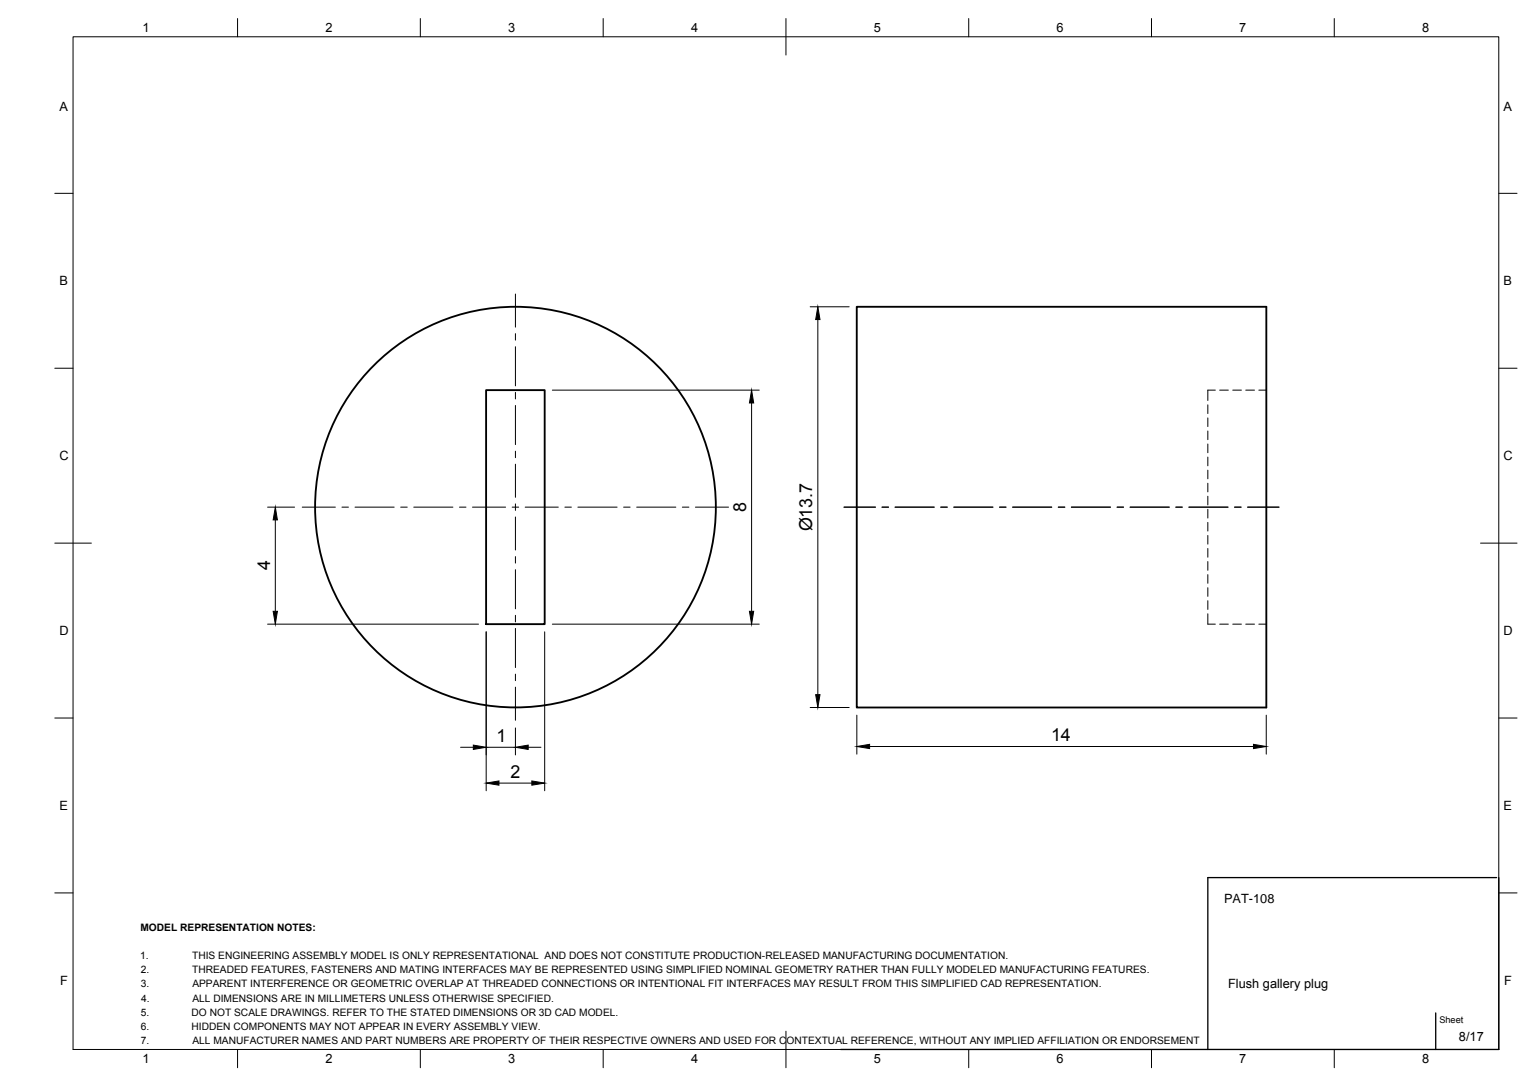
ISO-10303-21;
HEADER;
/* Generated by software containing ST-Developer
 * from STEP Tools, Inc. (www.steptools.com) 
 */

FILE_DESCRIPTION(
/* description */ ('Sub-base valve envelopes and connections'),
/* implementation_level */ '2;1');

FILE_NAME(
/* name */ 'Flush gallery plug.step',
/* time_stamp */ '2026-10-29T15:55:44-07:00',
/* author */ (''),
/* organization */ (''),
/* preprocessor_version */ 'ST-DEVELOPER v20.2',
/* originating_system */ 'Autodesk Translation Framework v15.17.0.0',
/* authorisation */ '');

FILE_SCHEMA (('AUTOMOTIVE_DESIGN { 1 0 10303 214 3 1 1 }'));
ENDSEC;

DATA;
#10=MECHANICAL_DESIGN_GEOMETRIC_PRESENTATION_REPRESENTATION('',(#124),#6113);
#100=SHAPE_REPRESENTATION_RELATIONSHIP('SRR','None',#6173,#112);
#112=ADVANCED_BREP_SHAPE_REPRESENTATION('',(#136),#6104);
#124=STYLED_ITEM('',(#6329),#136);
#136=MANIFOLD_SOLID_BREP('Body1',#3363);
#211=FACE_BOUND('',#762,.T.);
#326=PLANE('',#3711);
#327=PLANE('',#3712);
#328=PLANE('',#3713);
#329=PLANE('',#3714);
#330=PLANE('',#3715);
#331=PLANE('',#3716);
#332=PLANE('',#3720);
#488=FACE_OUTER_BOUND('',#756,.T.);
#489=FACE_OUTER_BOUND('',#757,.T.);
#490=FACE_OUTER_BOUND('',#758,.T.);
#491=FACE_OUTER_BOUND('',#759,.T.);
#492=FACE_OUTER_BOUND('',#760,.T.);
#493=FACE_OUTER_BOUND('',#761,.T.);
#494=FACE_OUTER_BOUND('',#763,.T.);
#495=FACE_OUTER_BOUND('',#764,.T.);
#756=EDGE_LOOP('',(#2681,#2682,#2683,#2684));
#757=EDGE_LOOP('',(#2685,#2686,#2687,#2688));
#758=EDGE_LOOP('',(#2689,#2690,#2691,#2692));
#759=EDGE_LOOP('',(#2693,#2694,#2695,#2696));
#760=EDGE_LOOP('',(#2697,#2698,#2699,#2700));
#761=EDGE_LOOP('',(#2701));
#762=EDGE_LOOP('',(#2702,#2703,#2704,#2705));
#763=EDGE_LOOP('',(#2706,#2707,#2708,#2709));
#764=EDGE_LOOP('',(#2710));
#1008=LINE('',#5634,#1242);
#1009=LINE('',#5636,#1243);
#1010=LINE('',#5638,#1244);
#1011=LINE('',#5639,#1245);
#1012=LINE('',#5642,#1246);
#1013=LINE('',#5644,#1247);
#1014=LINE('',#5645,#1248);
#1015=LINE('',#5648,#1249);
#1016=LINE('',#5650,#1250);
#1017=LINE('',#5651,#1251);
#1018=LINE('',#5653,#1252);
#1019=LINE('',#5654,#1253);
#1020=LINE('',#5661,#1254);
#1242=VECTOR('',#4428,1.);
#1243=VECTOR('',#4429,1.);
#1244=VECTOR('',#4430,1.);
#1245=VECTOR('',#4431,1.);
#1246=VECTOR('',#4434,1.);
#1247=VECTOR('',#4435,1.);
#1248=VECTOR('',#4436,1.);
#1249=VECTOR('',#4439,1.);
#1250=VECTOR('',#4440,1.);
#1251=VECTOR('',#4441,1.);
#1252=VECTOR('',#4444,1.);
#1253=VECTOR('',#4445,1.);
#1254=VECTOR('',#4454,0.685);
#1467=CIRCLE('',#3717,0.685);
#1468=CIRCLE('',#3719,0.685);
#1685=VERTEX_POINT('',#5632);
#1686=VERTEX_POINT('',#5633);
#1687=VERTEX_POINT('',#5635);
#1688=VERTEX_POINT('',#5637);
#1689=VERTEX_POINT('',#5641);
#1690=VERTEX_POINT('',#5643);
#1691=VERTEX_POINT('',#5647);
#1692=VERTEX_POINT('',#5649);
#1693=VERTEX_POINT('',#5657);
#1694=VERTEX_POINT('',#5660);
#2038=EDGE_CURVE('',#1685,#1686,#1008,.T.);
#2039=EDGE_CURVE('',#1687,#1685,#1009,.T.);
#2040=EDGE_CURVE('',#1688,#1687,#1010,.T.);
#2041=EDGE_CURVE('',#1688,#1686,#1011,.T.);
#2042=EDGE_CURVE('',#1686,#1689,#1012,.T.);
#2043=EDGE_CURVE('',#1690,#1688,#1013,.T.);
#2044=EDGE_CURVE('',#1690,#1689,#1014,.T.);
#2045=EDGE_CURVE('',#1689,#1691,#1015,.T.);
#2046=EDGE_CURVE('',#1692,#1690,#1016,.T.);
#2047=EDGE_CURVE('',#1692,#1691,#1017,.T.);
#2048=EDGE_CURVE('',#1691,#1685,#1018,.T.);
#2049=EDGE_CURVE('',#1687,#1692,#1019,.T.);
#2050=EDGE_CURVE('',#1693,#1693,#1467,.T.);
#2051=EDGE_CURVE('',#1693,#1694,#1020,.T.);
#2052=EDGE_CURVE('',#1694,#1694,#1468,.T.);
#2681=ORIENTED_EDGE('',*,*,#2038,.F.);
#2682=ORIENTED_EDGE('',*,*,#2039,.F.);
#2683=ORIENTED_EDGE('',*,*,#2040,.F.);
#2684=ORIENTED_EDGE('',*,*,#2041,.T.);
#2685=ORIENTED_EDGE('',*,*,#2042,.F.);
#2686=ORIENTED_EDGE('',*,*,#2041,.F.);
#2687=ORIENTED_EDGE('',*,*,#2043,.F.);
#2688=ORIENTED_EDGE('',*,*,#2044,.T.);
#2689=ORIENTED_EDGE('',*,*,#2045,.F.);
#2690=ORIENTED_EDGE('',*,*,#2044,.F.);
#2691=ORIENTED_EDGE('',*,*,#2046,.F.);
#2692=ORIENTED_EDGE('',*,*,#2047,.T.);
#2693=ORIENTED_EDGE('',*,*,#2048,.F.);
#2694=ORIENTED_EDGE('',*,*,#2047,.F.);
#2695=ORIENTED_EDGE('',*,*,#2049,.F.);
#2696=ORIENTED_EDGE('',*,*,#2039,.T.);
#2697=ORIENTED_EDGE('',*,*,#2043,.T.);
#2698=ORIENTED_EDGE('',*,*,#2040,.T.);
#2699=ORIENTED_EDGE('',*,*,#2049,.T.);
#2700=ORIENTED_EDGE('',*,*,#2046,.T.);
#2701=ORIENTED_EDGE('',*,*,#2050,.T.);
#2702=ORIENTED_EDGE('',*,*,#2045,.T.);
#2703=ORIENTED_EDGE('',*,*,#2048,.T.);
#2704=ORIENTED_EDGE('',*,*,#2038,.T.);
#2705=ORIENTED_EDGE('',*,*,#2042,.T.);
#2706=ORIENTED_EDGE('',*,*,#2050,.F.);
#2707=ORIENTED_EDGE('',*,*,#2051,.T.);
#2708=ORIENTED_EDGE('',*,*,#2052,.T.);
#2709=ORIENTED_EDGE('',*,*,#2051,.F.);
#2710=ORIENTED_EDGE('',*,*,#2052,.F.);
#3126=CYLINDRICAL_SURFACE('',#3718,0.685);
#3261=ADVANCED_FACE('',(#488),#326,.F.);
#3262=ADVANCED_FACE('',(#489),#327,.F.);
#3263=ADVANCED_FACE('',(#490),#328,.F.);
#3264=ADVANCED_FACE('',(#491),#329,.F.);
#3265=ADVANCED_FACE('',(#492),#330,.T.);
#3266=ADVANCED_FACE('',(#493,#211),#331,.T.);
#3267=ADVANCED_FACE('',(#494),#3126,.T.);
#3268=ADVANCED_FACE('',(#495),#332,.F.);
#3363=CLOSED_SHELL('',(#3261,#3262,#3263,#3264,#3265,#3266,#3267,#3268));
#3710=AXIS2_PLACEMENT_3D('',#5630,#4424,#4425);
#3711=AXIS2_PLACEMENT_3D('',#5631,#4426,#4427);
#3712=AXIS2_PLACEMENT_3D('',#5640,#4432,#4433);
#3713=AXIS2_PLACEMENT_3D('',#5646,#4437,#4438);
#3714=AXIS2_PLACEMENT_3D('',#5652,#4442,#4443);
#3715=AXIS2_PLACEMENT_3D('',#5655,#4446,#4447);
#3716=AXIS2_PLACEMENT_3D('',#5656,#4448,#4449);
#3717=AXIS2_PLACEMENT_3D('',#5658,#4450,#4451);
#3718=AXIS2_PLACEMENT_3D('',#5659,#4452,#4453);
#3719=AXIS2_PLACEMENT_3D('',#5662,#4455,#4456);
#3720=AXIS2_PLACEMENT_3D('',#5663,#4457,#4458);
#4424=DIRECTION('axis',(0.,0.,1.));
#4425=DIRECTION('refdir',(1.,0.,0.));
#4426=DIRECTION('center_axis',(0.,0.,-1.));
#4427=DIRECTION('ref_axis',(0.,1.,0.));
#4428=DIRECTION('',(0.,-1.,0.));
#4429=DIRECTION('',(1.,0.,0.));
#4430=DIRECTION('',(0.,1.,0.));
#4431=DIRECTION('',(1.,0.,0.));
#4432=DIRECTION('center_axis',(0.,-1.,0.));
#4433=DIRECTION('ref_axis',(0.,0.,-1.));
#4434=DIRECTION('',(0.,0.,1.));
#4435=DIRECTION('',(0.,0.,-1.));
#4436=DIRECTION('',(1.,0.,0.));
#4437=DIRECTION('center_axis',(0.,0.,1.));
#4438=DIRECTION('ref_axis',(0.,-1.,0.));
#4439=DIRECTION('',(0.,1.,0.));
#4440=DIRECTION('',(0.,-1.,0.));
#4441=DIRECTION('',(1.,0.,0.));
#4442=DIRECTION('center_axis',(0.,1.,0.));
#4443=DIRECTION('ref_axis',(0.,0.,1.));
#4444=DIRECTION('',(0.,0.,-1.));
#4445=DIRECTION('',(0.,0.,1.));
#4446=DIRECTION('center_axis',(1.,0.,0.));
#4447=DIRECTION('ref_axis',(0.,0.,-1.));
#4448=DIRECTION('center_axis',(1.,0.,0.));
#4449=DIRECTION('ref_axis',(0.,0.,-1.));
#4450=DIRECTION('center_axis',(1.,0.,0.));
#4451=DIRECTION('ref_axis',(0.,0.,-1.));
#4452=DIRECTION('center_axis',(1.,0.,0.));
#4453=DIRECTION('ref_axis',(0.,0.,-1.));
#4454=DIRECTION('',(-1.,0.,0.));
#4455=DIRECTION('center_axis',(1.,0.,0.));
#4456=DIRECTION('ref_axis',(0.,0.,-1.));
#4457=DIRECTION('center_axis',(1.,0.,0.));
#4458=DIRECTION('ref_axis',(0.,0.,-1.));
#5630=CARTESIAN_POINT('',(0.,0.,0.));
#5631=CARTESIAN_POINT('Origin',(5.3,-0.4,3.4));
#5632=CARTESIAN_POINT('',(5.5,0.4,3.4));
#5633=CARTESIAN_POINT('',(5.5,-0.4,3.4));
#5634=CARTESIAN_POINT('',(5.5,-0.2,3.4));
#5635=CARTESIAN_POINT('',(5.3,0.4,3.4));
#5636=CARTESIAN_POINT('',(5.3,0.4,3.4));
#5637=CARTESIAN_POINT('',(5.3,-0.4,3.4));
#5638=CARTESIAN_POINT('',(5.3,-0.4,3.4));
#5639=CARTESIAN_POINT('',(5.3,-0.4,3.4));
#5640=CARTESIAN_POINT('Origin',(5.3,-0.4,3.6));
#5641=CARTESIAN_POINT('',(5.5,-0.4,3.6));
#5642=CARTESIAN_POINT('',(5.5,-0.4,3.55));
#5643=CARTESIAN_POINT('',(5.3,-0.4,3.6));
#5644=CARTESIAN_POINT('',(5.3,-0.4,3.6));
#5645=CARTESIAN_POINT('',(5.3,-0.4,3.6));
#5646=CARTESIAN_POINT('Origin',(5.3,0.4,3.6));
#5647=CARTESIAN_POINT('',(5.5,0.4,3.6));
#5648=CARTESIAN_POINT('',(5.5,0.2,3.6));
#5649=CARTESIAN_POINT('',(5.3,0.4,3.6));
#5650=CARTESIAN_POINT('',(5.3,0.4,3.6));
#5651=CARTESIAN_POINT('',(5.3,0.4,3.6));
#5652=CARTESIAN_POINT('Origin',(5.3,0.4,3.4));
#5653=CARTESIAN_POINT('',(5.5,0.4,3.45));
#5654=CARTESIAN_POINT('',(5.3,0.4,3.4));
#5655=CARTESIAN_POINT('Origin',(5.3,0.,3.5));
#5656=CARTESIAN_POINT('Origin',(5.5,0.,3.5));
#5657=CARTESIAN_POINT('',(5.5,-8.38883057415937E-17,4.185));
#5658=CARTESIAN_POINT('Origin',(5.5,0.,3.5));
#5659=CARTESIAN_POINT('Origin',(4.1,0.,3.5));
#5660=CARTESIAN_POINT('',(4.1,-8.38883057415937E-17,4.185));
#5661=CARTESIAN_POINT('',(4.1,-8.38883057415937E-17,4.185));
#5662=CARTESIAN_POINT('Origin',(4.1,0.,3.5));
#5663=CARTESIAN_POINT('Origin',(4.1,0.,3.5));
#6088=UNCERTAINTY_MEASURE_WITH_UNIT(LENGTH_MEASURE(0.001),#6114,
'DISTANCE_ACCURACY_VALUE',
'Maximum model space distance between geometric entities at asserted c
onnectivities');
#6097=UNCERTAINTY_MEASURE_WITH_UNIT(LENGTH_MEASURE(0.001),#6114,
'DISTANCE_ACCURACY_VALUE',
'Maximum model space distance between geometric entities at asserted c
onnectivities');
#6104=(
GEOMETRIC_REPRESENTATION_CONTEXT(3)
GLOBAL_UNCERTAINTY_ASSIGNED_CONTEXT((#6088))
GLOBAL_UNIT_ASSIGNED_CONTEXT((#6114,#6116,#6117))
REPRESENTATION_CONTEXT('','3D')
);
#6113=(
GEOMETRIC_REPRESENTATION_CONTEXT(3)
GLOBAL_UNCERTAINTY_ASSIGNED_CONTEXT((#6097))
GLOBAL_UNIT_ASSIGNED_CONTEXT((#6114,#6116,#6117))
REPRESENTATION_CONTEXT('','3D')
);
#6114=(
LENGTH_UNIT()
NAMED_UNIT(*)
SI_UNIT(.CENTI.,.METRE.)
);
#6116=(
NAMED_UNIT(*)
PLANE_ANGLE_UNIT()
SI_UNIT($,.RADIAN.)
);
#6117=(
NAMED_UNIT(*)
SI_UNIT($,.STERADIAN.)
SOLID_ANGLE_UNIT()
);
#6124=SHAPE_DEFINITION_REPRESENTATION(#6139,#6173);
#6139=PRODUCT_DEFINITION_SHAPE('',$,#6189);
#6173=SHAPE_REPRESENTATION('',(#3710),#6104);
#6182=PRODUCT_DEFINITION_CONTEXT('part definition',#6229,'design');
#6189=PRODUCT_DEFINITION('Flush gallery plug','Flush gallery plug',
#6204,#6182);
#6204=PRODUCT_DEFINITION_FORMATION('',$,#6237);
#6229=APPLICATION_CONTEXT(
'Core Data for Automotive Mechanical Design Process');
#6230=PRODUCT_CONTEXT('part definition',#6229,'mechanical');
#6237=PRODUCT('Flush gallery plug','Flush gallery plug',
'Flush gallery plug',(#6230));
#6323=COLOUR_RGB('Off White',0.89,0.88,0.83);
#6324=FILL_AREA_STYLE_COLOUR('',#6323);
#6325=FILL_AREA_STYLE('',(#6324));
#6326=SURFACE_STYLE_FILL_AREA(#6325);
#6327=SURFACE_SIDE_STYLE('',(#6326));
#6328=SURFACE_STYLE_USAGE(.BOTH.,#6327);
#6329=PRESENTATION_STYLE_ASSIGNMENT((#6328));
ENDSEC;
END-ISO-10303-21;
